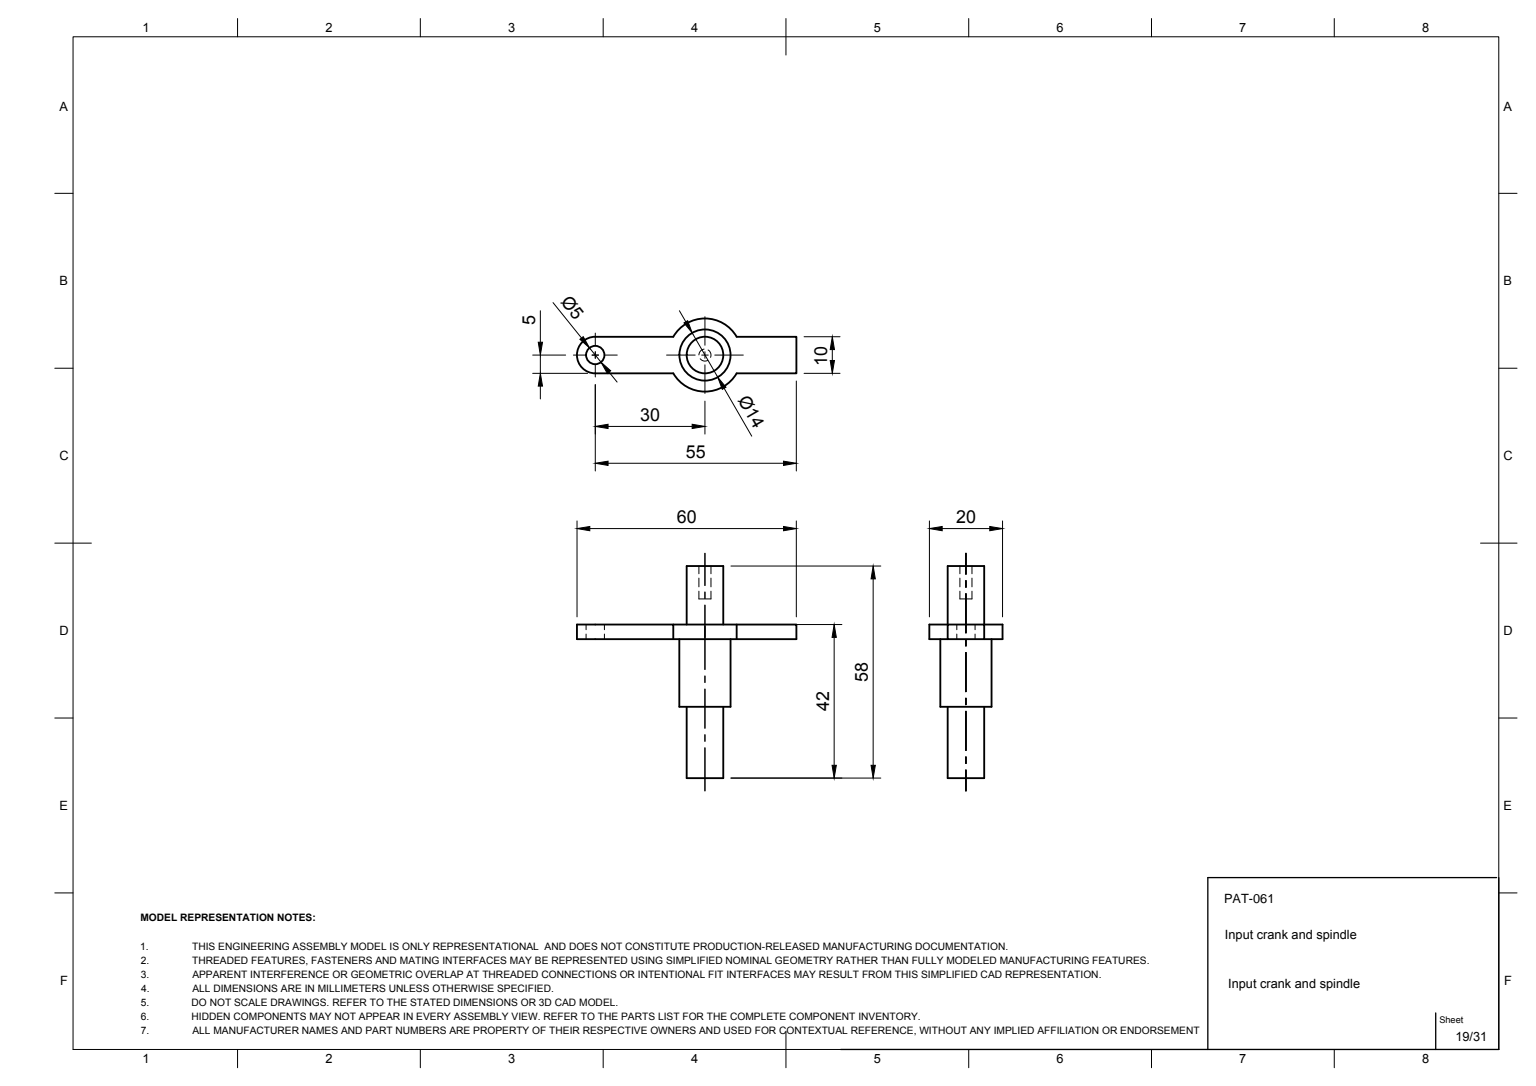
ISO-10303-21;
HEADER;
/* Generated by software containing ST-Developer
 * from STEP Tools, Inc. (www.steptools.com) 
 */

FILE_DESCRIPTION(
/* description */ ('Compact intermittent indexer'),
/* implementation_level */ '2;1');

FILE_NAME(
/* name */ 'Input crank and spindle.step',
/* time_stamp */ '2026-10-29T16:32:17-07:00',
/* author */ (''),
/* organization */ (''),
/* preprocessor_version */ 'ST-DEVELOPER v20.2',
/* originating_system */ 'Autodesk Translation Framework v15.17.0.0',
/* authorisation */ '');

FILE_SCHEMA (('AUTOMOTIVE_DESIGN { 1 0 10303 214 3 1 1 }'));
ENDSEC;

DATA;
#10=MECHANICAL_DESIGN_GEOMETRIC_PRESENTATION_REPRESENTATION('',(#276),#10837);
#220=SHAPE_REPRESENTATION_RELATIONSHIP('SRR','None',#10956,#244);
#244=ADVANCED_BREP_SHAPE_REPRESENTATION('',(#307),#10823);
#276=STYLED_ITEM('',(#11159),#307);
#307=MANIFOLD_SOLID_BREP('Body1',#5649);
#432=FACE_BOUND('',#1241,.T.);
#433=FACE_BOUND('',#1242,.T.);
#434=FACE_BOUND('',#1249,.T.);
#435=FACE_BOUND('',#1250,.T.);
#436=FACE_BOUND('',#1254,.T.);
#437=FACE_BOUND('',#1259,.T.);
#556=PLANE('',#6327);
#557=PLANE('',#6334);
#558=PLANE('',#6338);
#559=PLANE('',#6339);
#560=PLANE('',#6340);
#561=PLANE('',#6341);
#562=PLANE('',#6342);
#563=PLANE('',#6343);
#564=PLANE('',#6349);
#565=PLANE('',#6357);
#566=PLANE('',#6358);
#829=FACE_OUTER_BOUND('',#1236,.T.);
#830=FACE_OUTER_BOUND('',#1237,.T.);
#831=FACE_OUTER_BOUND('',#1238,.T.);
#832=FACE_OUTER_BOUND('',#1239,.T.);
#833=FACE_OUTER_BOUND('',#1240,.T.);
#834=FACE_OUTER_BOUND('',#1243,.T.);
#835=FACE_OUTER_BOUND('',#1244,.T.);
#836=FACE_OUTER_BOUND('',#1245,.T.);
#837=FACE_OUTER_BOUND('',#1246,.T.);
#838=FACE_OUTER_BOUND('',#1247,.T.);
#839=FACE_OUTER_BOUND('',#1248,.T.);
#840=FACE_OUTER_BOUND('',#1251,.T.);
#841=FACE_OUTER_BOUND('',#1252,.T.);
#842=FACE_OUTER_BOUND('',#1253,.T.);
#843=FACE_OUTER_BOUND('',#1255,.T.);
#844=FACE_OUTER_BOUND('',#1256,.T.);
#845=FACE_OUTER_BOUND('',#1257,.T.);
#846=FACE_OUTER_BOUND('',#1258,.T.);
#847=FACE_OUTER_BOUND('',#1260,.T.);
#1236=EDGE_LOOP('',(#4440,#4441,#4442,#4443));
#1237=EDGE_LOOP('',(#4444));
#1238=EDGE_LOOP('',(#4445,#4446,#4447,#4448));
#1239=EDGE_LOOP('',(#4449,#4450,#4451,#4452));
#1240=EDGE_LOOP('',(#4453,#4454,#4455,#4456,#4457,#4458,#4459,#4460));
#1241=EDGE_LOOP('',(#4461));
#1242=EDGE_LOOP('',(#4462));
#1243=EDGE_LOOP('',(#4463,#4464,#4465,#4466));
#1244=EDGE_LOOP('',(#4467,#4468,#4469,#4470));
#1245=EDGE_LOOP('',(#4471,#4472,#4473,#4474));
#1246=EDGE_LOOP('',(#4475,#4476,#4477,#4478));
#1247=EDGE_LOOP('',(#4479,#4480,#4481,#4482));
#1248=EDGE_LOOP('',(#4483,#4484,#4485,#4486,#4487,#4488,#4489,#4490));
#1249=EDGE_LOOP('',(#4491));
#1250=EDGE_LOOP('',(#4492));
#1251=EDGE_LOOP('',(#4493,#4494,#4495,#4496));
#1252=EDGE_LOOP('',(#4497,#4498,#4499,#4500));
#1253=EDGE_LOOP('',(#4501));
#1254=EDGE_LOOP('',(#4502));
#1255=EDGE_LOOP('',(#4503,#4504,#4505,#4506));
#1256=EDGE_LOOP('',(#4507,#4508,#4509,#4510));
#1257=EDGE_LOOP('',(#4511,#4512,#4513,#4514));
#1258=EDGE_LOOP('',(#4515));
#1259=EDGE_LOOP('',(#4516));
#1260=EDGE_LOOP('',(#4517));
#1580=LINE('',#9724,#1938);
#1581=LINE('',#9731,#1939);
#1582=LINE('',#9736,#1940);
#1583=LINE('',#9740,#1941);
#1584=LINE('',#9744,#1942);
#1585=LINE('',#9748,#1943);
#1586=LINE('',#9750,#1944);
#1587=LINE('',#9752,#1945);
#1588=LINE('',#9755,#1946);
#1589=LINE('',#9760,#1947);
#1590=LINE('',#9761,#1948);
#1591=LINE('',#9764,#1949);
#1592=LINE('',#9765,#1950);
#1593=LINE('',#9768,#1951);
#1594=LINE('',#9770,#1952);
#1595=LINE('',#9771,#1953);
#1596=LINE('',#9774,#1954);
#1597=LINE('',#9776,#1955);
#1598=LINE('',#9777,#1956);
#1599=LINE('',#9779,#1957);
#1600=LINE('',#9793,#1958);
#1601=LINE('',#9796,#1959);
#1602=LINE('',#9801,#1960);
#1938=VECTOR('',#7610,0.165);
#1939=VECTOR('',#7619,0.25);
#1940=VECTOR('',#7624,1.);
#1941=VECTOR('',#7627,1.);
#1942=VECTOR('',#7632,1.);
#1943=VECTOR('',#7635,1.);
#1944=VECTOR('',#7636,1.);
#1945=VECTOR('',#7637,1.);
#1946=VECTOR('',#7640,1.);
#1947=VECTOR('',#7645,1.);
#1948=VECTOR('',#7646,1.);
#1949=VECTOR('',#7649,1.);
#1950=VECTOR('',#7650,1.);
#1951=VECTOR('',#7653,1.);
#1952=VECTOR('',#7654,1.);
#1953=VECTOR('',#7655,1.);
#1954=VECTOR('',#7658,1.);
#1955=VECTOR('',#7659,1.);
#1956=VECTOR('',#7660,1.);
#1957=VECTOR('',#7663,1.);
#1958=VECTOR('',#7684,0.7);
#1959=VECTOR('',#7687,0.5);
#1960=VECTOR('',#7694,0.5);
#2346=CIRCLE('',#6325,0.165);
#2347=CIRCLE('',#6326,0.165);
#2348=CIRCLE('',#6329,0.25);
#2349=CIRCLE('',#6330,0.25);
#2350=CIRCLE('',#6332,0.5);
#2351=CIRCLE('',#6333,0.5);
#2352=CIRCLE('',#6335,1.);
#2353=CIRCLE('',#6336,1.);
#2354=CIRCLE('',#6337,0.7);
#2355=CIRCLE('',#6344,1.);
#2356=CIRCLE('',#6345,1.);
#2357=CIRCLE('',#6346,0.5);
#2358=CIRCLE('',#6350,0.7);
#2359=CIRCLE('',#6351,0.5);
#2360=CIRCLE('',#6354,0.5);
#2361=CIRCLE('',#6356,0.5);
#2734=VERTEX_POINT('',#9721);
#2735=VERTEX_POINT('',#9723);
#2736=VERTEX_POINT('',#9728);
#2737=VERTEX_POINT('',#9730);
#2738=VERTEX_POINT('',#9734);
#2739=VERTEX_POINT('',#9735);
#2740=VERTEX_POINT('',#9737);
#2741=VERTEX_POINT('',#9739);
#2742=VERTEX_POINT('',#9743);
#2743=VERTEX_POINT('',#9745);
#2744=VERTEX_POINT('',#9747);
#2745=VERTEX_POINT('',#9749);
#2746=VERTEX_POINT('',#9751);
#2747=VERTEX_POINT('',#9753);
#2748=VERTEX_POINT('',#9756);
#2749=VERTEX_POINT('',#9759);
#2750=VERTEX_POINT('',#9763);
#2751=VERTEX_POINT('',#9767);
#2752=VERTEX_POINT('',#9769);
#2753=VERTEX_POINT('',#9773);
#2754=VERTEX_POINT('',#9775);
#2755=VERTEX_POINT('',#9783);
#2756=VERTEX_POINT('',#9788);
#2757=VERTEX_POINT('',#9790);
#2758=VERTEX_POINT('',#9795);
#2759=VERTEX_POINT('',#9799);
#3342=EDGE_CURVE('',#2734,#2734,#2346,.T.);
#3343=EDGE_CURVE('',#2734,#2735,#1580,.T.);
#3344=EDGE_CURVE('',#2735,#2735,#2347,.T.);
#3345=EDGE_CURVE('',#2736,#2736,#2348,.T.);
#3346=EDGE_CURVE('',#2736,#2737,#1581,.T.);
#3347=EDGE_CURVE('',#2737,#2737,#2349,.T.);
#3348=EDGE_CURVE('',#2738,#2739,#1582,.T.);
#3349=EDGE_CURVE('',#2740,#2739,#2350,.T.);
#3350=EDGE_CURVE('',#2741,#2740,#1583,.T.);
#3351=EDGE_CURVE('',#2741,#2738,#2351,.T.);
#3352=EDGE_CURVE('',#2742,#2741,#1584,.T.);
#3353=EDGE_CURVE('',#2743,#2742,#2352,.T.);
#3354=EDGE_CURVE('',#2744,#2743,#1585,.T.);
#3355=EDGE_CURVE('',#2745,#2744,#1586,.T.);
#3356=EDGE_CURVE('',#2746,#2745,#1587,.T.);
#3357=EDGE_CURVE('',#2747,#2746,#2353,.T.);
#3358=EDGE_CURVE('',#2738,#2747,#1588,.T.);
#3359=EDGE_CURVE('',#2748,#2748,#2354,.T.);
#3360=EDGE_CURVE('',#2749,#2747,#1589,.T.);
#3361=EDGE_CURVE('',#2739,#2749,#1590,.T.);
#3362=EDGE_CURVE('',#2742,#2750,#1591,.T.);
#3363=EDGE_CURVE('',#2750,#2740,#1592,.T.);
#3364=EDGE_CURVE('',#2751,#2743,#1593,.T.);
#3365=EDGE_CURVE('',#2752,#2751,#1594,.T.);
#3366=EDGE_CURVE('',#2744,#2752,#1595,.T.);
#3367=EDGE_CURVE('',#2746,#2753,#1596,.T.);
#3368=EDGE_CURVE('',#2745,#2754,#1597,.T.);
#3369=EDGE_CURVE('',#2753,#2754,#1598,.T.);
#3370=EDGE_CURVE('',#2754,#2752,#1599,.T.);
#3371=EDGE_CURVE('',#2749,#2753,#2355,.T.);
#3372=EDGE_CURVE('',#2751,#2750,#2356,.T.);
#3373=EDGE_CURVE('',#2755,#2755,#2357,.T.);
#3374=EDGE_CURVE('',#2756,#2756,#2358,.T.);
#3375=EDGE_CURVE('',#2757,#2757,#2359,.T.);
#3376=EDGE_CURVE('',#2748,#2756,#1600,.T.);
#3377=EDGE_CURVE('',#2757,#2758,#1601,.T.);
#3378=EDGE_CURVE('',#2758,#2758,#2360,.T.);
#3379=EDGE_CURVE('',#2759,#2759,#2361,.T.);
#3380=EDGE_CURVE('',#2759,#2755,#1602,.T.);
#4440=ORIENTED_EDGE('',*,*,#3342,.F.);
#4441=ORIENTED_EDGE('',*,*,#3343,.T.);
#4442=ORIENTED_EDGE('',*,*,#3344,.F.);
#4443=ORIENTED_EDGE('',*,*,#3343,.F.);
#4444=ORIENTED_EDGE('',*,*,#3342,.T.);
#4445=ORIENTED_EDGE('',*,*,#3345,.F.);
#4446=ORIENTED_EDGE('',*,*,#3346,.T.);
#4447=ORIENTED_EDGE('',*,*,#3347,.F.);
#4448=ORIENTED_EDGE('',*,*,#3346,.F.);
#4449=ORIENTED_EDGE('',*,*,#3348,.T.);
#4450=ORIENTED_EDGE('',*,*,#3349,.F.);
#4451=ORIENTED_EDGE('',*,*,#3350,.F.);
#4452=ORIENTED_EDGE('',*,*,#3351,.T.);
#4453=ORIENTED_EDGE('',*,*,#3352,.F.);
#4454=ORIENTED_EDGE('',*,*,#3353,.F.);
#4455=ORIENTED_EDGE('',*,*,#3354,.F.);
#4456=ORIENTED_EDGE('',*,*,#3355,.F.);
#4457=ORIENTED_EDGE('',*,*,#3356,.F.);
#4458=ORIENTED_EDGE('',*,*,#3357,.F.);
#4459=ORIENTED_EDGE('',*,*,#3358,.F.);
#4460=ORIENTED_EDGE('',*,*,#3351,.F.);
#4461=ORIENTED_EDGE('',*,*,#3345,.T.);
#4462=ORIENTED_EDGE('',*,*,#3359,.T.);
#4463=ORIENTED_EDGE('',*,*,#3360,.F.);
#4464=ORIENTED_EDGE('',*,*,#3361,.F.);
#4465=ORIENTED_EDGE('',*,*,#3348,.F.);
#4466=ORIENTED_EDGE('',*,*,#3358,.T.);
#4467=ORIENTED_EDGE('',*,*,#3362,.F.);
#4468=ORIENTED_EDGE('',*,*,#3352,.T.);
#4469=ORIENTED_EDGE('',*,*,#3350,.T.);
#4470=ORIENTED_EDGE('',*,*,#3363,.F.);
#4471=ORIENTED_EDGE('',*,*,#3364,.F.);
#4472=ORIENTED_EDGE('',*,*,#3365,.F.);
#4473=ORIENTED_EDGE('',*,*,#3366,.F.);
#4474=ORIENTED_EDGE('',*,*,#3354,.T.);
#4475=ORIENTED_EDGE('',*,*,#3367,.F.);
#4476=ORIENTED_EDGE('',*,*,#3356,.T.);
#4477=ORIENTED_EDGE('',*,*,#3368,.T.);
#4478=ORIENTED_EDGE('',*,*,#3369,.F.);
#4479=ORIENTED_EDGE('',*,*,#3355,.T.);
#4480=ORIENTED_EDGE('',*,*,#3366,.T.);
#4481=ORIENTED_EDGE('',*,*,#3370,.F.);
#4482=ORIENTED_EDGE('',*,*,#3368,.F.);
#4483=ORIENTED_EDGE('',*,*,#3361,.T.);
#4484=ORIENTED_EDGE('',*,*,#3371,.T.);
#4485=ORIENTED_EDGE('',*,*,#3369,.T.);
#4486=ORIENTED_EDGE('',*,*,#3370,.T.);
#4487=ORIENTED_EDGE('',*,*,#3365,.T.);
#4488=ORIENTED_EDGE('',*,*,#3372,.T.);
#4489=ORIENTED_EDGE('',*,*,#3363,.T.);
#4490=ORIENTED_EDGE('',*,*,#3349,.T.);
#4491=ORIENTED_EDGE('',*,*,#3347,.T.);
#4492=ORIENTED_EDGE('',*,*,#3373,.F.);
#4493=ORIENTED_EDGE('',*,*,#3364,.T.);
#4494=ORIENTED_EDGE('',*,*,#3353,.T.);
#4495=ORIENTED_EDGE('',*,*,#3362,.T.);
#4496=ORIENTED_EDGE('',*,*,#3372,.F.);
#4497=ORIENTED_EDGE('',*,*,#3367,.T.);
#4498=ORIENTED_EDGE('',*,*,#3371,.F.);
#4499=ORIENTED_EDGE('',*,*,#3360,.T.);
#4500=ORIENTED_EDGE('',*,*,#3357,.T.);
#4501=ORIENTED_EDGE('',*,*,#3374,.F.);
#4502=ORIENTED_EDGE('',*,*,#3375,.F.);
#4503=ORIENTED_EDGE('',*,*,#3359,.F.);
#4504=ORIENTED_EDGE('',*,*,#3376,.T.);
#4505=ORIENTED_EDGE('',*,*,#3374,.T.);
#4506=ORIENTED_EDGE('',*,*,#3376,.F.);
#4507=ORIENTED_EDGE('',*,*,#3375,.T.);
#4508=ORIENTED_EDGE('',*,*,#3377,.T.);
#4509=ORIENTED_EDGE('',*,*,#3378,.T.);
#4510=ORIENTED_EDGE('',*,*,#3377,.F.);
#4511=ORIENTED_EDGE('',*,*,#3379,.F.);
#4512=ORIENTED_EDGE('',*,*,#3380,.T.);
#4513=ORIENTED_EDGE('',*,*,#3373,.T.);
#4514=ORIENTED_EDGE('',*,*,#3380,.F.);
#4515=ORIENTED_EDGE('',*,*,#3379,.T.);
#4516=ORIENTED_EDGE('',*,*,#3344,.T.);
#4517=ORIENTED_EDGE('',*,*,#3378,.F.);
#5238=CYLINDRICAL_SURFACE('',#6324,0.165);
#5239=CYLINDRICAL_SURFACE('',#6328,0.25);
#5240=CYLINDRICAL_SURFACE('',#6331,0.5);
#5241=CYLINDRICAL_SURFACE('',#6347,1.);
#5242=CYLINDRICAL_SURFACE('',#6348,1.);
#5243=CYLINDRICAL_SURFACE('',#6352,0.7);
#5244=CYLINDRICAL_SURFACE('',#6353,0.5);
#5245=CYLINDRICAL_SURFACE('',#6355,0.5);
#5472=ADVANCED_FACE('',(#829),#5238,.F.);
#5473=ADVANCED_FACE('',(#830),#556,.T.);
#5474=ADVANCED_FACE('',(#831),#5239,.F.);
#5475=ADVANCED_FACE('',(#832),#5240,.T.);
#5476=ADVANCED_FACE('',(#833,#432,#433),#557,.F.);
#5477=ADVANCED_FACE('',(#834),#558,.T.);
#5478=ADVANCED_FACE('',(#835),#559,.T.);
#5479=ADVANCED_FACE('',(#836),#560,.T.);
#5480=ADVANCED_FACE('',(#837),#561,.T.);
#5481=ADVANCED_FACE('',(#838),#562,.T.);
#5482=ADVANCED_FACE('',(#839,#434,#435),#563,.T.);
#5483=ADVANCED_FACE('',(#840),#5241,.T.);
#5484=ADVANCED_FACE('',(#841),#5242,.T.);
#5485=ADVANCED_FACE('',(#842,#436),#564,.F.);
#5486=ADVANCED_FACE('',(#843),#5243,.T.);
#5487=ADVANCED_FACE('',(#844),#5244,.T.);
#5488=ADVANCED_FACE('',(#845),#5245,.T.);
#5489=ADVANCED_FACE('',(#846,#437),#565,.T.);
#5490=ADVANCED_FACE('',(#847),#566,.F.);
#5649=CLOSED_SHELL('',(#5472,#5473,#5474,#5475,#5476,#5477,#5478,#5479,
#5480,#5481,#5482,#5483,#5484,#5485,#5486,#5487,#5488,#5489,#5490));
#6323=AXIS2_PLACEMENT_3D('',#9719,#7604,#7605);
#6324=AXIS2_PLACEMENT_3D('',#9720,#7606,#7607);
#6325=AXIS2_PLACEMENT_3D('',#9722,#7608,#7609);
#6326=AXIS2_PLACEMENT_3D('',#9725,#7611,#7612);
#6327=AXIS2_PLACEMENT_3D('',#9726,#7613,#7614);
#6328=AXIS2_PLACEMENT_3D('',#9727,#7615,#7616);
#6329=AXIS2_PLACEMENT_3D('',#9729,#7617,#7618);
#6330=AXIS2_PLACEMENT_3D('',#9732,#7620,#7621);
#6331=AXIS2_PLACEMENT_3D('',#9733,#7622,#7623);
#6332=AXIS2_PLACEMENT_3D('',#9738,#7625,#7626);
#6333=AXIS2_PLACEMENT_3D('',#9741,#7628,#7629);
#6334=AXIS2_PLACEMENT_3D('',#9742,#7630,#7631);
#6335=AXIS2_PLACEMENT_3D('',#9746,#7633,#7634);
#6336=AXIS2_PLACEMENT_3D('',#9754,#7638,#7639);
#6337=AXIS2_PLACEMENT_3D('',#9757,#7641,#7642);
#6338=AXIS2_PLACEMENT_3D('',#9758,#7643,#7644);
#6339=AXIS2_PLACEMENT_3D('',#9762,#7647,#7648);
#6340=AXIS2_PLACEMENT_3D('',#9766,#7651,#7652);
#6341=AXIS2_PLACEMENT_3D('',#9772,#7656,#7657);
#6342=AXIS2_PLACEMENT_3D('',#9778,#7661,#7662);
#6343=AXIS2_PLACEMENT_3D('',#9780,#7664,#7665);
#6344=AXIS2_PLACEMENT_3D('',#9781,#7666,#7667);
#6345=AXIS2_PLACEMENT_3D('',#9782,#7668,#7669);
#6346=AXIS2_PLACEMENT_3D('',#9784,#7670,#7671);
#6347=AXIS2_PLACEMENT_3D('',#9785,#7672,#7673);
#6348=AXIS2_PLACEMENT_3D('',#9786,#7674,#7675);
#6349=AXIS2_PLACEMENT_3D('',#9787,#7676,#7677);
#6350=AXIS2_PLACEMENT_3D('',#9789,#7678,#7679);
#6351=AXIS2_PLACEMENT_3D('',#9791,#7680,#7681);
#6352=AXIS2_PLACEMENT_3D('',#9792,#7682,#7683);
#6353=AXIS2_PLACEMENT_3D('',#9794,#7685,#7686);
#6354=AXIS2_PLACEMENT_3D('',#9797,#7688,#7689);
#6355=AXIS2_PLACEMENT_3D('',#9798,#7690,#7691);
#6356=AXIS2_PLACEMENT_3D('',#9800,#7692,#7693);
#6357=AXIS2_PLACEMENT_3D('',#9802,#7695,#7696);
#6358=AXIS2_PLACEMENT_3D('',#9803,#7697,#7698);
#7604=DIRECTION('axis',(0.,0.,1.));
#7605=DIRECTION('refdir',(1.,0.,0.));
#7606=DIRECTION('center_axis',(0.,0.,1.));
#7607=DIRECTION('ref_axis',(1.,0.,0.));
#7608=DIRECTION('center_axis',(0.,0.,1.));
#7609=DIRECTION('ref_axis',(1.,0.,0.));
#7610=DIRECTION('',(0.,0.,1.));
#7611=DIRECTION('center_axis',(0.,0.,-1.));
#7612=DIRECTION('ref_axis',(1.,0.,0.));
#7613=DIRECTION('center_axis',(0.,0.,1.));
#7614=DIRECTION('ref_axis',(1.,0.,0.));
#7615=DIRECTION('center_axis',(0.,0.,1.));
#7616=DIRECTION('ref_axis',(1.,0.,0.));
#7617=DIRECTION('center_axis',(0.,0.,1.));
#7618=DIRECTION('ref_axis',(1.,0.,0.));
#7619=DIRECTION('',(0.,0.,1.));
#7620=DIRECTION('center_axis',(0.,0.,-1.));
#7621=DIRECTION('ref_axis',(1.,0.,0.));
#7622=DIRECTION('center_axis',(0.,0.,1.));
#7623=DIRECTION('ref_axis',(1.,0.,0.));
#7624=DIRECTION('',(0.,0.,1.));
#7625=DIRECTION('center_axis',(0.,0.,1.));
#7626=DIRECTION('ref_axis',(1.,0.,0.));
#7627=DIRECTION('',(0.,0.,1.));
#7628=DIRECTION('center_axis',(0.,0.,1.));
#7629=DIRECTION('ref_axis',(1.,0.,0.));
#7630=DIRECTION('center_axis',(0.,0.,1.));
#7631=DIRECTION('ref_axis',(1.,0.,0.));
#7632=DIRECTION('',(1.,0.,0.));
#7633=DIRECTION('center_axis',(0.,0.,1.));
#7634=DIRECTION('ref_axis',(1.,0.,0.));
#7635=DIRECTION('',(1.,0.,0.));
#7636=DIRECTION('',(0.,-1.,0.));
#7637=DIRECTION('',(-1.,0.,0.));
#7638=DIRECTION('center_axis',(0.,0.,1.));
#7639=DIRECTION('ref_axis',(1.,0.,0.));
#7640=DIRECTION('',(-1.,0.,0.));
#7641=DIRECTION('center_axis',(0.,0.,1.));
#7642=DIRECTION('ref_axis',(1.,0.,0.));
#7643=DIRECTION('center_axis',(0.,1.,0.));
#7644=DIRECTION('ref_axis',(-1.,0.,0.));
#7645=DIRECTION('',(0.,0.,-1.));
#7646=DIRECTION('',(-1.,0.,0.));
#7647=DIRECTION('center_axis',(0.,-1.,0.));
#7648=DIRECTION('ref_axis',(1.,0.,0.));
#7649=DIRECTION('',(0.,0.,1.));
#7650=DIRECTION('',(1.,0.,0.));
#7651=DIRECTION('center_axis',(0.,-1.,0.));
#7652=DIRECTION('ref_axis',(1.,0.,0.));
#7653=DIRECTION('',(0.,0.,-1.));
#7654=DIRECTION('',(1.,0.,0.));
#7655=DIRECTION('',(0.,0.,1.));
#7656=DIRECTION('center_axis',(0.,1.,0.));
#7657=DIRECTION('ref_axis',(-1.,0.,0.));
#7658=DIRECTION('',(0.,0.,1.));
#7659=DIRECTION('',(0.,0.,1.));
#7660=DIRECTION('',(-1.,0.,0.));
#7661=DIRECTION('center_axis',(-1.,0.,0.));
#7662=DIRECTION('ref_axis',(0.,-1.,0.));
#7663=DIRECTION('',(0.,-1.,0.));
#7664=DIRECTION('center_axis',(0.,0.,1.));
#7665=DIRECTION('ref_axis',(1.,0.,0.));
#7666=DIRECTION('center_axis',(0.,0.,1.));
#7667=DIRECTION('ref_axis',(1.,0.,0.));
#7668=DIRECTION('center_axis',(0.,0.,1.));
#7669=DIRECTION('ref_axis',(1.,0.,0.));
#7670=DIRECTION('center_axis',(0.,0.,1.));
#7671=DIRECTION('ref_axis',(1.,0.,0.));
#7672=DIRECTION('center_axis',(0.,0.,1.));
#7673=DIRECTION('ref_axis',(1.,0.,0.));
#7674=DIRECTION('center_axis',(0.,0.,1.));
#7675=DIRECTION('ref_axis',(1.,0.,0.));
#7676=DIRECTION('center_axis',(0.,0.,1.));
#7677=DIRECTION('ref_axis',(1.,0.,0.));
#7678=DIRECTION('center_axis',(0.,0.,1.));
#7679=DIRECTION('ref_axis',(1.,0.,0.));
#7680=DIRECTION('center_axis',(0.,0.,-1.));
#7681=DIRECTION('ref_axis',(1.,0.,0.));
#7682=DIRECTION('center_axis',(0.,0.,1.));
#7683=DIRECTION('ref_axis',(1.,0.,0.));
#7684=DIRECTION('',(0.,0.,-1.));
#7685=DIRECTION('center_axis',(0.,0.,1.));
#7686=DIRECTION('ref_axis',(1.,0.,0.));
#7687=DIRECTION('',(0.,0.,-1.));
#7688=DIRECTION('center_axis',(0.,0.,1.));
#7689=DIRECTION('ref_axis',(1.,0.,0.));
#7690=DIRECTION('center_axis',(0.,0.,1.));
#7691=DIRECTION('ref_axis',(1.,0.,0.));
#7692=DIRECTION('center_axis',(0.,0.,1.));
#7693=DIRECTION('ref_axis',(1.,0.,0.));
#7694=DIRECTION('',(0.,0.,-1.));
#7695=DIRECTION('center_axis',(0.,0.,1.));
#7696=DIRECTION('ref_axis',(1.,0.,0.));
#7697=DIRECTION('center_axis',(0.,0.,1.));
#7698=DIRECTION('ref_axis',(1.,0.,0.));
#9719=CARTESIAN_POINT('',(0.,0.,0.));
#9720=CARTESIAN_POINT('Origin',(0.,0.,5.9));
#9721=CARTESIAN_POINT('',(-0.165,-2.02066721859313E-17,5.9));
#9722=CARTESIAN_POINT('Origin',(0.,0.,5.9));
#9723=CARTESIAN_POINT('',(-0.165,2.02066721859313E-17,6.8));
#9724=CARTESIAN_POINT('',(-0.165,-2.02066721859313E-17,5.9));
#9725=CARTESIAN_POINT('Origin',(0.,0.,6.8));
#9726=CARTESIAN_POINT('Origin',(0.,0.,5.9));
#9727=CARTESIAN_POINT('Origin',(3.,0.,4.7));
#9728=CARTESIAN_POINT('',(2.75,-3.06161699786838E-17,4.8));
#9729=CARTESIAN_POINT('Origin',(3.,0.,4.8));
#9730=CARTESIAN_POINT('',(2.75,3.06161699786838E-17,5.2));
#9731=CARTESIAN_POINT('',(2.75,-3.06161699786838E-17,4.7));
#9732=CARTESIAN_POINT('Origin',(3.,0.,5.2));
#9733=CARTESIAN_POINT('Origin',(3.,0.,4.8));
#9734=CARTESIAN_POINT('',(3.,0.5,4.8));
#9735=CARTESIAN_POINT('',(3.,0.5,5.2));
#9736=CARTESIAN_POINT('',(3.,0.5,4.8));
#9737=CARTESIAN_POINT('',(3.,-0.5,5.2));
#9738=CARTESIAN_POINT('Origin',(3.,0.,5.2));
#9739=CARTESIAN_POINT('',(3.,-0.5,4.8));
#9740=CARTESIAN_POINT('',(3.,-0.5,4.8));
#9741=CARTESIAN_POINT('Origin',(3.,0.,4.8));
#9742=CARTESIAN_POINT('Origin',(0.,0.,4.8));
#9743=CARTESIAN_POINT('',(0.866025403784439,-0.5,4.8));
#9744=CARTESIAN_POINT('',(-2.5,-0.5,4.8));
#9745=CARTESIAN_POINT('',(-0.866025403784439,-0.5,4.8));
#9746=CARTESIAN_POINT('Origin',(0.,0.,4.8));
#9747=CARTESIAN_POINT('',(-2.5,-0.5,4.8));
#9748=CARTESIAN_POINT('',(-2.5,-0.5,4.8));
#9749=CARTESIAN_POINT('',(-2.5,0.5,4.8));
#9750=CARTESIAN_POINT('',(-2.5,0.5,4.8));
#9751=CARTESIAN_POINT('',(-0.866025403784439,0.5,4.8));
#9752=CARTESIAN_POINT('',(3.,0.5,4.8));
#9753=CARTESIAN_POINT('',(0.866025403784439,0.5,4.8));
#9754=CARTESIAN_POINT('Origin',(0.,0.,4.8));
#9755=CARTESIAN_POINT('',(3.,0.5,4.8));
#9756=CARTESIAN_POINT('',(-0.7,-8.57252759403147E-17,4.8));
#9757=CARTESIAN_POINT('Origin',(0.,0.,4.8));
#9758=CARTESIAN_POINT('Origin',(3.,0.5,4.8));
#9759=CARTESIAN_POINT('',(0.866025403784439,0.5,5.2));
#9760=CARTESIAN_POINT('',(0.866025403784439,0.5,4.8));
#9761=CARTESIAN_POINT('',(3.,0.5,5.2));
#9762=CARTESIAN_POINT('Origin',(-2.5,-0.5,4.8));
#9763=CARTESIAN_POINT('',(0.866025403784439,-0.5,5.2));
#9764=CARTESIAN_POINT('',(0.866025403784439,-0.5,4.8));
#9765=CARTESIAN_POINT('',(-2.5,-0.5,5.2));
#9766=CARTESIAN_POINT('Origin',(-2.5,-0.5,4.8));
#9767=CARTESIAN_POINT('',(-0.866025403784439,-0.5,5.2));
#9768=CARTESIAN_POINT('',(-0.866025403784439,-0.5,4.8));
#9769=CARTESIAN_POINT('',(-2.5,-0.5,5.2));
#9770=CARTESIAN_POINT('',(-2.5,-0.5,5.2));
#9771=CARTESIAN_POINT('',(-2.5,-0.5,4.8));
#9772=CARTESIAN_POINT('Origin',(3.,0.5,4.8));
#9773=CARTESIAN_POINT('',(-0.866025403784439,0.5,5.2));
#9774=CARTESIAN_POINT('',(-0.866025403784439,0.5,4.8));
#9775=CARTESIAN_POINT('',(-2.5,0.5,5.2));
#9776=CARTESIAN_POINT('',(-2.5,0.5,4.8));
#9777=CARTESIAN_POINT('',(3.,0.5,5.2));
#9778=CARTESIAN_POINT('Origin',(-2.5,0.5,4.8));
#9779=CARTESIAN_POINT('',(-2.5,0.5,5.2));
#9780=CARTESIAN_POINT('Origin',(0.,0.,5.2));
#9781=CARTESIAN_POINT('Origin',(0.,0.,5.2));
#9782=CARTESIAN_POINT('Origin',(0.,0.,5.2));
#9783=CARTESIAN_POINT('',(-0.5,-6.12323399573677E-17,5.2));
#9784=CARTESIAN_POINT('Origin',(0.,0.,5.2));
#9785=CARTESIAN_POINT('Origin',(0.,0.,4.8));
#9786=CARTESIAN_POINT('Origin',(0.,0.,4.8));
#9787=CARTESIAN_POINT('Origin',(0.,0.,2.95));
#9788=CARTESIAN_POINT('',(-0.7,-8.57252759403147E-17,2.95));
#9789=CARTESIAN_POINT('Origin',(0.,0.,2.95));
#9790=CARTESIAN_POINT('',(-0.5,6.12323399573677E-17,2.95));
#9791=CARTESIAN_POINT('Origin',(0.,0.,2.95));
#9792=CARTESIAN_POINT('Origin',(0.,0.,2.95));
#9793=CARTESIAN_POINT('',(-0.7,-8.57252759403147E-17,2.95));
#9794=CARTESIAN_POINT('Origin',(0.,0.,1.));
#9795=CARTESIAN_POINT('',(-0.5,-6.12323399573677E-17,1.));
#9796=CARTESIAN_POINT('',(-0.5,-6.12323399573677E-17,1.));
#9797=CARTESIAN_POINT('Origin',(0.,0.,1.));
#9798=CARTESIAN_POINT('Origin',(0.,0.,1.));
#9799=CARTESIAN_POINT('',(-0.5,-6.12323399573677E-17,6.8));
#9800=CARTESIAN_POINT('Origin',(0.,0.,6.8));
#9801=CARTESIAN_POINT('',(-0.5,-6.12323399573677E-17,1.));
#9802=CARTESIAN_POINT('Origin',(0.,0.,6.8));
#9803=CARTESIAN_POINT('Origin',(0.,0.,1.));
#10793=UNCERTAINTY_MEASURE_WITH_UNIT(LENGTH_MEASURE(0.001),#10838,
'DISTANCE_ACCURACY_VALUE',
'Maximum model space distance between geometric entities at asserted c
onnectivities');
#10807=UNCERTAINTY_MEASURE_WITH_UNIT(LENGTH_MEASURE(0.001),#10838,
'DISTANCE_ACCURACY_VALUE',
'Maximum model space distance between geometric entities at asserted c
onnectivities');
#10823=(
GEOMETRIC_REPRESENTATION_CONTEXT(3)
GLOBAL_UNCERTAINTY_ASSIGNED_CONTEXT((#10793))
GLOBAL_UNIT_ASSIGNED_CONTEXT((#10838,#10840,#10841))
REPRESENTATION_CONTEXT('','3D')
);
#10837=(
GEOMETRIC_REPRESENTATION_CONTEXT(3)
GLOBAL_UNCERTAINTY_ASSIGNED_CONTEXT((#10807))
GLOBAL_UNIT_ASSIGNED_CONTEXT((#10838,#10840,#10841))
REPRESENTATION_CONTEXT('','3D')
);
#10838=(
LENGTH_UNIT()
NAMED_UNIT(*)
SI_UNIT(.CENTI.,.METRE.)
);
#10840=(
NAMED_UNIT(*)
PLANE_ANGLE_UNIT()
SI_UNIT($,.RADIAN.)
);
#10841=(
NAMED_UNIT(*)
SI_UNIT($,.STERADIAN.)
SOLID_ANGLE_UNIT()
);
#10857=SHAPE_DEFINITION_REPRESENTATION(#10891,#10956);
#10891=PRODUCT_DEFINITION_SHAPE('',$,#10986);
#10956=SHAPE_REPRESENTATION('',(#6323),#10823);
#10970=PRODUCT_DEFINITION_CONTEXT('part definition',#11059,'design');
#10986=PRODUCT_DEFINITION('Input crank and spindle',
'Input crank and spindle',#11015,#10970);
#11015=PRODUCT_DEFINITION_FORMATION('',$,#11076);
#11059=APPLICATION_CONTEXT(
'Core Data for Automotive Mechanical Design Process');
#11060=PRODUCT_CONTEXT('part definition',#11059,'mechanical');
#11076=PRODUCT('Input crank and spindle','Input crank and spindle',
'Input crank and spindle',(#11060));
#11153=COLOUR_RGB('Sky Blue',0.24,0.69,0.87);
#11154=FILL_AREA_STYLE_COLOUR('',#11153);
#11155=FILL_AREA_STYLE('',(#11154));
#11156=SURFACE_STYLE_FILL_AREA(#11155);
#11157=SURFACE_SIDE_STYLE('',(#11156));
#11158=SURFACE_STYLE_USAGE(.BOTH.,#11157);
#11159=PRESENTATION_STYLE_ASSIGNMENT((#11158));
ENDSEC;
END-ISO-10303-21;
